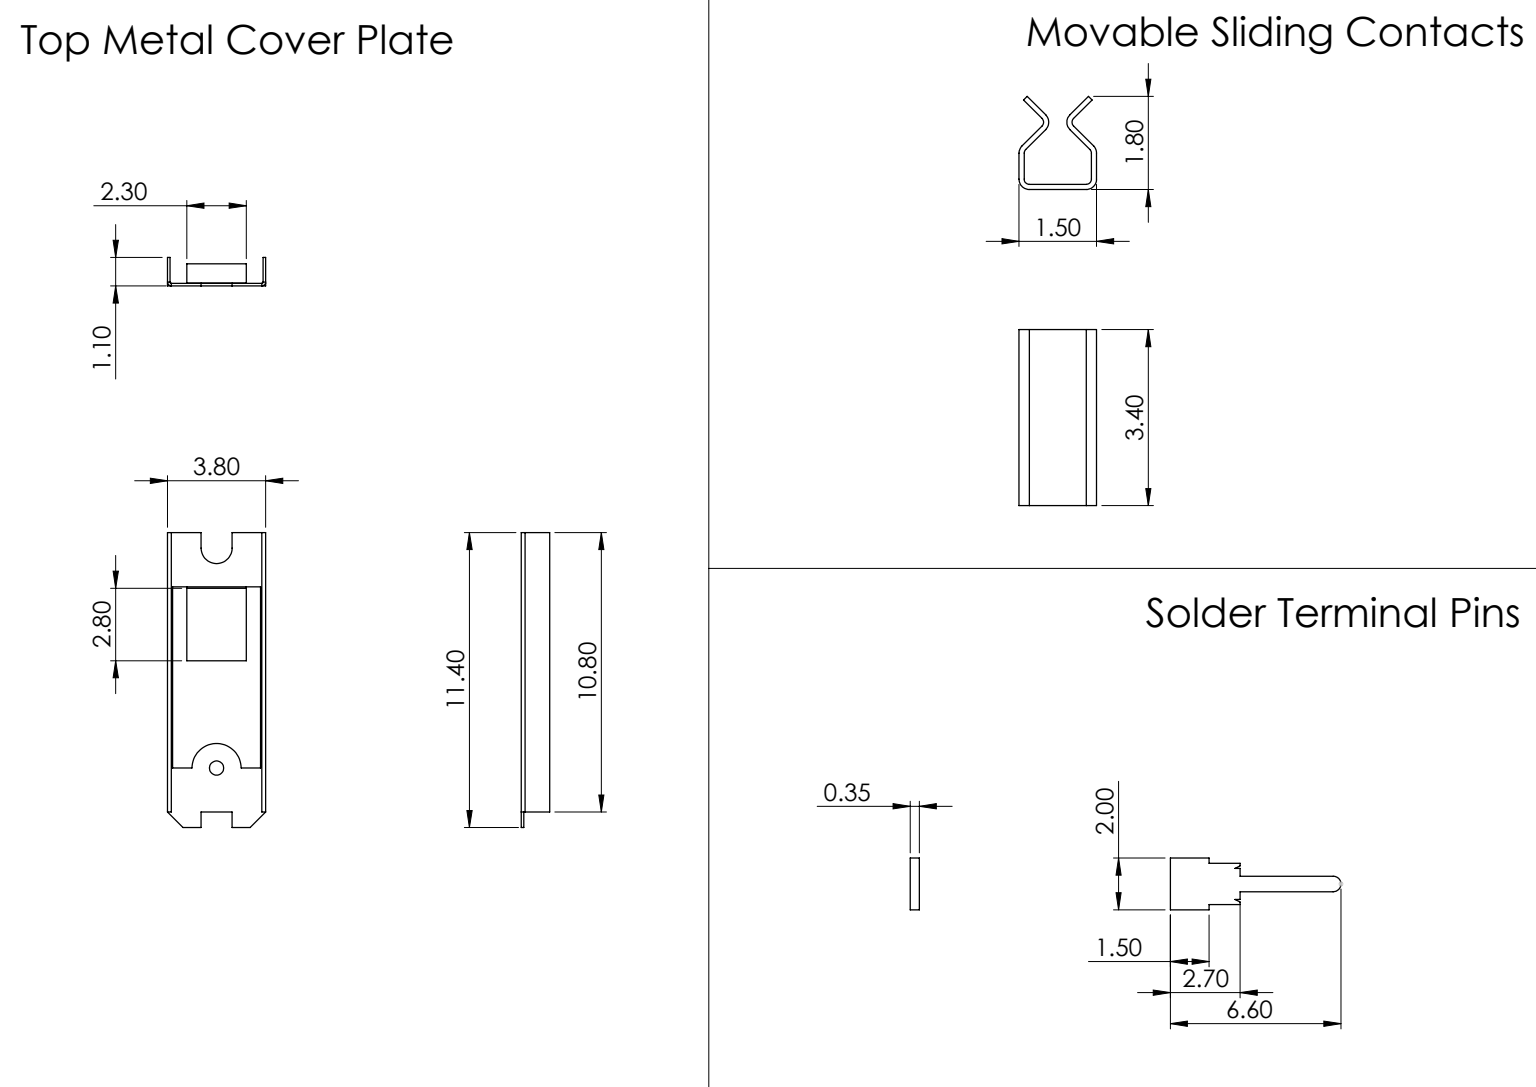
ISO-10303-21;
HEADER;
FILE_DESCRIPTION (('STEP AP214'),
    '1' );
FILE_NAME ('Solder Terminal Pins.step',
    '2026-10-09T19:32:29',
    ( '' ),
    ( '' ),
    'SwSTEP 2.0',
    'SolidWorks 2026',
    '' );
FILE_SCHEMA (( 'AUTOMOTIVE_DESIGN' ));
ENDSEC;

DATA;
#30=AXIS2_PLACEMENT_3D ( 'NONE', #13757, #16263, #2391 ) ;
#40=ORIENTED_EDGE ( 'NONE', *, *, #16715, .F. ) ;
#50=EDGE_LOOP ( 'NONE', ( #8387, #9597, #10554, #1667 ) ) ;
#66=ORIENTED_EDGE ( 'NONE', *, *, #5755, .T. ) ;
#103=VERTEX_POINT ( 'NONE', #12339 ) ;
#220=VECTOR ( 'NONE', #13007, 1000.000000000000000 ) ;
#244=APPLICATION_CONTEXT ( 'automotive_design' ) ;
#250=LINE ( 'NONE', #4404, #4362 ) ;
#296=CARTESIAN_POINT ( 'NONE',  ( 0.1749999999999999889, 8.800000000000000711, 0.4000000000000000222 ) ) ;
#310=ORIENTED_EDGE ( 'NONE', *, *, #13145, .F. ) ;
#326=ORIENTED_EDGE ( 'NONE', *, *, #6822, .T. ) ;
#331=VECTOR ( 'NONE', #11702, 1000.000000000000000 ) ;
#359=EDGE_CURVE ( 'NONE', #3082, #8454, #16331, .T. ) ;
#369=CARTESIAN_POINT ( 'NONE',  ( 0.1749999999999999889, 7.500000000000000000, 3.100000000000000089 ) ) ;
#450=VECTOR ( 'NONE', #504, 1000.000000000000000 ) ;
#504=DIRECTION ( 'NONE',  ( 5.551115123125779621E-17, 0.000000000000000000, 1.000000000000000000 ) ) ;
#537=CARTESIAN_POINT ( 'NONE',  ( -0.1749999999999999889, 8.200000000000001066, 0.4000000000000000222 ) ) ;
#551=DIRECTION ( 'NONE',  ( 0.000000000000000000, -1.000000000000000000, 0.000000000000000000 ) ) ;
#613=DIRECTION ( 'NONE',  ( 0.000000000000000000, 1.000000000000000000, 0.000000000000000000 ) ) ;
#646=CIRCLE ( 'NONE', #2745, 0.2999999999999999334 ) ;
#649=DIRECTION ( 'NONE',  ( -1.000000000000000000, 0.000000000000000000, 1.586032892321649771E-16 ) ) ;
#682=EDGE_CURVE ( 'NONE', #13202, #15500, #5739, .T. ) ;
#711=EDGE_CURVE ( 'NONE', #12486, #8493, #10165, .T. ) ;
#716=CARTESIAN_POINT ( 'NONE',  ( 0.1749999999999999889, 9.199999999999999289, 0.4000000000000000222 ) ) ;
#743=ORIENTED_EDGE ( 'NONE', *, *, #1591, .T. ) ;
#780=CARTESIAN_POINT ( 'NONE',  ( 0.1749999999999999889, 7.900000000000000355, 0.4000000000000000222 ) ) ;
#828=DIRECTION ( 'NONE',  ( 0.000000000000000000, 0.000000000000000000, -1.000000000000000000 ) ) ;
#853=SHAPE_REPRESENTATION ( 'Solder Terminal Pins', ( #17681 ), #4692 ) ;
#900=EDGE_LOOP ( 'NONE', ( #8185, #16443, #4602, #11112 ) ) ;
#904=FACE_OUTER_BOUND ( 'NONE', #4232, .T. ) ;
#915=CARTESIAN_POINT ( 'NONE',  ( 0.1749999999999999889, 9.500000000000000000, 3.100000000000000089 ) ) ;
#918=DIRECTION ( 'NONE',  ( -1.000000000000000000, 0.000000000000000000, 1.268826313857320014E-15 ) ) ;
#947=ADVANCED_FACE ( 'NONE', ( #4699 ), #14962, .T. ) ;
#953=ORIENTED_EDGE ( 'NONE', *, *, #17999, .F. ) ;
#959=VERTEX_POINT ( 'NONE', #2271 ) ;
#1067=FACE_OUTER_BOUND ( 'NONE', #7693, .T. ) ;
#1086=VECTOR ( 'NONE', #16477, 1000.000000000000000 ) ;
#1143=VECTOR ( 'NONE', #11238, 1000.000000000000000 ) ;
#1148=MECHANICAL_DESIGN_GEOMETRIC_PRESENTATION_REPRESENTATION('',(#6157),#4396);
#1164=PLANE ( 'NONE',  #16782 ) ;
#1218=PRODUCT_DEFINITION_CONTEXT ( 'detailed design', #244, 'design' ) ;
#1255=CARTESIAN_POINT ( 'NONE',  ( -0.1749999999999999889, 9.299999999999998934, 1.600000000000000089 ) ) ;
#1302=ORIENTED_EDGE ( 'NONE', *, *, #9005, .T. ) ;
#1311=CARTESIAN_POINT ( 'NONE',  ( -0.1749999999999999889, 7.700000000000000178, 1.600000000000000089 ) ) ;
#1333=DIRECTION ( 'NONE',  ( -6.167905692361979821E-17, 0.000000000000000000, -1.000000000000000000 ) ) ;
#1360=DIRECTION ( 'NONE',  ( -6.938893903907229610E-17, 0.000000000000000000, -1.000000000000000000 ) ) ;
#1389=VERTEX_POINT ( 'NONE', #15100 ) ;
#1403=CARTESIAN_POINT ( 'NONE',  ( -0.1749999999999999889, 8.200000000000001066, 0.4000000000000000222 ) ) ;
#1407=CARTESIAN_POINT ( 'NONE',  ( -0.1749999999999999889, 9.500000000000000000, 1.600000000000000089 ) ) ;
#1456=EDGE_LOOP ( 'NONE', ( #16915, #13820, #14175, #17317 ) ) ;
#1462=CARTESIAN_POINT ( 'NONE',  ( 0.1749999999999999889, 8.500000000000000000, -3.200000000000000178 ) ) ;
#1467=VECTOR ( 'NONE', #8980, 1000.000000000000000 ) ;
#1563=ORIENTED_EDGE ( 'NONE', *, *, #7259, .F. ) ;
#1568=ADVANCED_FACE ( 'NONE', ( #8498 ), #14148, .T. ) ;
#1591=EDGE_CURVE ( 'NONE', #4752, #1389, #4856, .T. ) ;
#1648=( LENGTH_UNIT ( ) NAMED_UNIT ( * ) SI_UNIT ( .MILLI., .METRE. ) );
#1667=ORIENTED_EDGE ( 'NONE', *, *, #711, .F. ) ;
#1669=ADVANCED_FACE ( 'NONE', ( #11908 ), #17176, .T. ) ;
#1693=ORIENTED_EDGE ( 'NONE', *, *, #17999, .T. ) ;
#1695=VECTOR ( 'NONE', #2486, 1000.000000000000114 ) ;
#1733=CARTESIAN_POINT ( 'NONE',  ( -0.1749999999999999889, 7.500000000000000000, 1.600000000000000089 ) ) ;
#1758=DIRECTION ( 'NONE',  ( -1.000000000000000000, 0.000000000000000000, 0.000000000000000000 ) ) ;
#1796=ORIENTED_EDGE ( 'NONE', *, *, #9182, .T. ) ;
#1803=CARTESIAN_POINT ( 'NONE',  ( -0.1749999999999999889, 7.799999999999999822, 0.4000000000000000222 ) ) ;
#1882=PLANE ( 'NONE',  #9376 ) ;
#1936=DIRECTION ( 'NONE',  ( 0.000000000000000000, 0.000000000000000000, -1.000000000000000000 ) ) ;
#1965=EDGE_LOOP ( 'NONE', ( #1302, #12791, #12438, #15138 ) ) ;
#2001=CARTESIAN_POINT ( 'NONE',  ( 0.1749999999999999889, 7.700000000000000178, 1.600000000000000089 ) ) ;
#2030=AXIS2_PLACEMENT_3D ( 'NONE', #6738, #13497, #12015 ) ;
#2031=LINE ( 'NONE', #13150, #5224 ) ;
#2052=VERTEX_POINT ( 'NONE', #11654 ) ;
#2094=ADVANCED_FACE ( 'NONE', ( #4882 ), #4704, .T. ) ;
#2101=LINE ( 'NONE', #9517, #11767 ) ;
#2139=CARTESIAN_POINT ( 'NONE',  ( -0.1749999999999999889, 9.199999999999999289, 0.4000000000000000222 ) ) ;
#2181=LINE ( 'NONE', #17608, #18254 ) ;
#2185=CARTESIAN_POINT ( 'NONE',  ( 0.1749999999999999889, 8.800000000000000711, -3.200000000000000178 ) ) ;
#2207=LINE ( 'NONE', #12020, #13126 ) ;
#2216=CARTESIAN_POINT ( 'NONE',  ( 0.1749999999999999889, 7.900000000000000355, 0.4000000000000000222 ) ) ;
#2232=LINE ( 'NONE', #13632, #3944 ) ;
#2271=CARTESIAN_POINT ( 'NONE',  ( 0.1749999999999999889, 9.500000000000000000, 3.100000000000000089 ) ) ;
#2273=DIRECTION ( 'NONE',  ( -1.000000000000000000, 0.000000000000000000, 0.000000000000000000 ) ) ;
#2345=VECTOR ( 'NONE', #6024, 1000.000000000000000 ) ;
#2391=DIRECTION ( 'NONE',  ( 0.000000000000000000, -1.000000000000000000, 0.000000000000000000 ) ) ;
#2414=EDGE_CURVE ( 'NONE', #11896, #13928, #2232, .T. ) ;
#2437=VERTEX_POINT ( 'NONE', #6771 ) ;
#2461=LINE ( 'NONE', #13744, #2914 ) ;
#2486=DIRECTION ( 'NONE',  ( 0.000000000000000000, -0.4472135954999567065, -0.8944271909999164105 ) ) ;
#2489=CARTESIAN_POINT ( 'NONE',  ( 0.1749999999999999889, 7.700000000000000178, 1.600000000000000089 ) ) ;
#2503=PLANE ( 'NONE',  #4069 ) ;
#2547=AXIS2_PLACEMENT_3D ( 'NONE', #17886, #15337, #3732 ) ;
#2567=LINE ( 'NONE', #16456, #17986 ) ;
#2569=EDGE_CURVE ( 'NONE', #8663, #9757, #2207, .T. ) ;
#2631=VECTOR ( 'NONE', #4875, 1000.000000000000000 ) ;
#2665=ORIENTED_EDGE ( 'NONE', *, *, #4156, .T. ) ;
#2745=AXIS2_PLACEMENT_3D ( 'NONE', #8071, #13711, #9339 ) ;
#2823=DIRECTION ( 'NONE',  ( 0.000000000000000000, -1.000000000000000000, 0.000000000000000000 ) ) ;
#2826=CARTESIAN_POINT ( 'NONE',  ( 0.1749999999999999889, 8.200000000000001066, 0.4000000000000000222 ) ) ;
#2834=CARTESIAN_POINT ( 'NONE',  ( 0.1749999999999999889, 9.500000000000000000, 1.600000000000000089 ) ) ;
#2914=VECTOR ( 'NONE', #5417, 1000.000000000000000 ) ;
#2920=ORIENTED_EDGE ( 'NONE', *, *, #5177, .T. ) ;
#2948=VERTEX_POINT ( 'NONE', #5196 ) ;
#2968=VECTOR ( 'NONE', #7672, 1000.000000000000000 ) ;
#3009=ORIENTED_EDGE ( 'NONE', *, *, #16003, .F. ) ;
#3015=ORIENTED_EDGE ( 'NONE', *, *, #9251, .T. ) ;
#3039=CARTESIAN_POINT ( 'NONE',  ( -0.1749999999999999889, 7.500000000000000000, 3.100000000000000089 ) ) ;
#3052=ADVANCED_FACE ( 'NONE', ( #5395 ), #11036, .T. ) ;
#3080=ORIENTED_EDGE ( 'NONE', *, *, #16715, .T. ) ;
#3081=LINE ( 'NONE', #5773, #1143 ) ;
#3082=VERTEX_POINT ( 'NONE', #1311 ) ;
#3092=CARTESIAN_POINT ( 'NONE',  ( 0.1749999999999999889, 7.700000000000000178, 0.4000000000000000222 ) ) ;
#3097=DIRECTION ( 'NONE',  ( 0.000000000000000000, -1.000000000000000000, 2.220446049250320181E-15 ) ) ;
#3108=ORIENTED_EDGE ( 'NONE', *, *, #16254, .F. ) ;
#3112=DIRECTION ( 'NONE',  ( -0.000000000000000000, 1.000000000000000000, 0.000000000000000000 ) ) ;
#3141=EDGE_CURVE ( 'NONE', #11906, #17304, #16772, .T. ) ;
#3300=ORIENTED_EDGE ( 'NONE', *, *, #9251, .F. ) ;
#3321=ORIENTED_EDGE ( 'NONE', *, *, #1591, .F. ) ;
#3325=PLANE ( 'NONE',  #10300 ) ;
#3402=CARTESIAN_POINT ( 'NONE',  ( -0.1749999999999999889, 8.800000000000000711, -3.200000000000000178 ) ) ;
#3415=CARTESIAN_POINT ( 'NONE',  ( 0.1749999999999999889, 9.099999999999999645, 0.4000000000000000222 ) ) ;
#3502=ORIENTED_EDGE ( 'NONE', *, *, #4388, .F. ) ;
#3506=VERTEX_POINT ( 'NONE', #2185 ) ;
#3517=ORIENTED_EDGE ( 'NONE', *, *, #5755, .F. ) ;
#3581=CARTESIAN_POINT ( 'NONE',  ( -0.1749999999999999889, 7.799999999999999822, 0.4000000000000000222 ) ) ;
#3597=CARTESIAN_POINT ( 'NONE',  ( 0.1749999999999999889, 7.700000000000000178, 0.4000000000000000222 ) ) ;
#3609=PLANE ( 'NONE',  #10566 ) ;
#3732=DIRECTION ( 'NONE',  ( 1.000000000000000000, 0.000000000000000000, 0.000000000000000000 ) ) ;
#3764=AXIS2_PLACEMENT_3D ( 'NONE', #16684, #6873, #14935 ) ;
#3812=LINE ( 'NONE', #6385, #11862 ) ;
#3831=DIRECTION ( 'NONE',  ( 0.000000000000000000, -1.000000000000000000, 0.000000000000000000 ) ) ;
#3867=LINE ( 'NONE', #3581, #4101 ) ;
#3874=FACE_OUTER_BOUND ( 'NONE', #13904, .T. ) ;
#3876=ORIENTED_EDGE ( 'NONE', *, *, #12580, .F. ) ;
#3924=FACE_OUTER_BOUND ( 'NONE', #11029, .T. ) ;
#3925=PLANE ( 'NONE',  #2547 ) ;
#3944=VECTOR ( 'NONE', #15120, 1000.000000000000000 ) ;
#4012=FACE_OUTER_BOUND ( 'NONE', #5869, .T. ) ;
#4069=AXIS2_PLACEMENT_3D ( 'NONE', #12224, #12136, #14814 ) ;
#4101=VECTOR ( 'NONE', #10628, 1000.000000000000000 ) ;
#4146=DIRECTION ( 'NONE',  ( 1.000000000000000000, 0.000000000000000000, 0.000000000000000000 ) ) ;
#4156=EDGE_CURVE ( 'NONE', #8493, #13928, #15310, .T. ) ;
#4159=CARTESIAN_POINT ( 'NONE',  ( 0.1749999999999999889, 7.799999999999999822, 0.4000000000000000222 ) ) ;
#4207=CARTESIAN_POINT ( 'NONE',  ( -0.1749999999999999889, 9.099999999999999645, 0.4000000000000000222 ) ) ;
#4222=CARTESIAN_POINT ( 'NONE',  ( 0.1749999999999999889, 8.800000000000000711, 0.4000000000000000222 ) ) ;
#4232=EDGE_LOOP ( 'NONE', ( #15122, #5278, #8292, #15026, #9377, #4506, #743, #9277, #4667, #10100, #2665, #17005, #5084, #11412, #1796, #2920, #6120, #18045 ) ) ;
#4256=AXIS2_PLACEMENT_3D ( 'NONE', #10529, #10355, #4985 ) ;
#4307=EDGE_CURVE ( 'NONE', #13650, #6378, #2031, .T. ) ;
#4311=DIRECTION ( 'NONE',  ( -1.000000000000000000, -9.028005242978079560E-48, 6.123233995736769734E-17 ) ) ;
#4347=AXIS2_PLACEMENT_3D ( 'NONE', #7837, #10710, #6726 ) ;
#4362=VECTOR ( 'NONE', #5889, 1000.000000000000000 ) ;
#4388=EDGE_CURVE ( 'NONE', #17710, #103, #12973, .T. ) ;
#4396=( GEOMETRIC_REPRESENTATION_CONTEXT ( 3 ) GLOBAL_UNCERTAINTY_ASSIGNED_CONTEXT ( ( #5299 ) ) GLOBAL_UNIT_ASSIGNED_CONTEXT ( ( #13099, #4837, #14651 ) ) REPRESENTATION_CONTEXT ( 'NONE', 'WORKASPACE' ) );
#4401=CARTESIAN_POINT ( 'NONE',  ( 0.1749999999999999889, 8.200000000000001066, -3.200000000000000178 ) ) ;
#4404=CARTESIAN_POINT ( 'NONE',  ( -0.1749999999999999889, 7.900000000000000355, 0.4000000000000000222 ) ) ;
#4441=CIRCLE ( 'NONE', #5631, 0.2999999999999999334 ) ;
#4470=DIRECTION ( 'NONE',  ( 6.938893903907229610E-17, 0.000000000000000000, 1.000000000000000000 ) ) ;
#4496=CARTESIAN_POINT ( 'NONE',  ( -0.1749999999999999889, 9.099999999999999645, 0.5999999999999999778 ) ) ;
#4506=ORIENTED_EDGE ( 'NONE', *, *, #5071, .T. ) ;
#4518=LINE ( 'NONE', #369, #2968 ) ;
#4554=CARTESIAN_POINT ( 'NONE',  ( 0.1749999999999999889, 9.299999999999998934, 0.4000000000000000222 ) ) ;
#4559=FILL_AREA_STYLE ('',( #15792 ) ) ;
#4568=CARTESIAN_POINT ( 'NONE',  ( 0.1749999999999999889, 7.799999999999999822, 0.4000000000000000222 ) ) ;
#4570=EDGE_CURVE ( 'NONE', #9728, #8493, #646, .T. ) ;
#4602=ORIENTED_EDGE ( 'NONE', *, *, #12870, .F. ) ;
#4615=PLANE ( 'NONE',  #6400 ) ;
#4667=ORIENTED_EDGE ( 'NONE', *, *, #15207, .T. ) ;
#4672=LINE ( 'NONE', #8934, #450 ) ;
#4692=( GEOMETRIC_REPRESENTATION_CONTEXT ( 3 ) GLOBAL_UNCERTAINTY_ASSIGNED_CONTEXT ( ( #9735 ) ) GLOBAL_UNIT_ASSIGNED_CONTEXT ( ( #1648, #11831, #15812 ) ) REPRESENTATION_CONTEXT ( 'NONE', 'WORKASPACE' ) );
#4699=FACE_OUTER_BOUND ( 'NONE', #15626, .T. ) ;
#4704=PLANE ( 'NONE',  #4256 ) ;
#4752=VERTEX_POINT ( 'NONE', #9901 ) ;
#4788=ORIENTED_EDGE ( 'NONE', *, *, #12474, .F. ) ;
#4807=VERTEX_POINT ( 'NONE', #780 ) ;
#4820=EDGE_CURVE ( 'NONE', #13610, #2948, #4672, .T. ) ;
#4837=( NAMED_UNIT ( * ) PLANE_ANGLE_UNIT ( ) SI_UNIT ( $, .RADIAN. ) );
#4856=LINE ( 'NONE', #4496, #15202 ) ;
#4875=DIRECTION ( 'NONE',  ( 0.000000000000000000, -1.000000000000000000, 0.000000000000000000 ) ) ;
#4882=FACE_OUTER_BOUND ( 'NONE', #900, .T. ) ;
#4899=DIRECTION ( 'NONE',  ( 0.000000000000000000, -0.4472135954999631458, 0.8944271909999133019 ) ) ;
#4917=VECTOR ( 'NONE', #14522, 1000.000000000000000 ) ;
#4972=AXIS2_PLACEMENT_3D ( 'NONE', #12151, #9355, #12576 ) ;
#4978=VECTOR ( 'NONE', #918, 1000.000000000000000 ) ;
#4985=DIRECTION ( 'NONE',  ( 1.000000000000000000, 0.000000000000000000, 0.000000000000000000 ) ) ;
#5045=ADVANCED_FACE ( 'NONE', ( #4012 ), #3925, .T. ) ;
#5071=EDGE_CURVE ( 'NONE', #6378, #4752, #2461, .T. ) ;
#5084=ORIENTED_EDGE ( 'NONE', *, *, #7259, .T. ) ;
#5099=AXIS2_PLACEMENT_3D ( 'NONE', #14607, #10698, #1758 ) ;
#5165=PLANE ( 'NONE',  #7988 ) ;
#5177=EDGE_CURVE ( 'NONE', #5929, #3082, #7182, .T. ) ;
#5191=LINE ( 'NONE', #3415, #15640 ) ;
#5196=CARTESIAN_POINT ( 'NONE',  ( 0.1749999999999999889, 7.500000000000000000, 3.100000000000000089 ) ) ;
#5224=VECTOR ( 'NONE', #16030, 1000.000000000000000 ) ;
#5230=ORIENTED_EDGE ( 'NONE', *, *, #15207, .F. ) ;
#5269=DIRECTION ( 'NONE',  ( 0.000000000000000000, 0.000000000000000000, -1.000000000000000000 ) ) ;
#5278=ORIENTED_EDGE ( 'NONE', *, *, #17844, .T. ) ;
#5299=UNCERTAINTY_MEASURE_WITH_UNIT (LENGTH_MEASURE( 1.000000000000000082E-05 ), #13099, 'distance_accuracy_value', 'NONE');
#5320=LINE ( 'NONE', #10966, #17668 ) ;
#5386=ORIENTED_EDGE ( 'NONE', *, *, #682, .T. ) ;
#5395=FACE_OUTER_BOUND ( 'NONE', #6299, .T. ) ;
#5417=DIRECTION ( 'NONE',  ( 0.000000000000000000, -0.4472135954999631458, 0.8944271909999133019 ) ) ;
#5434=DIRECTION ( 'NONE',  ( 0.000000000000000000, -0.4472135954999567065, -0.8944271909999164105 ) ) ;
#5469=EDGE_LOOP ( 'NONE', ( #7657, #8304, #15068, #310 ) ) ;
#5490=CARTESIAN_POINT ( 'NONE',  ( 0.1749999999999999889, 9.299999999999998934, 1.600000000000000089 ) ) ;
#5556=VECTOR ( 'NONE', #5656, 1000.000000000000000 ) ;
#5594=VECTOR ( 'NONE', #6045, 1000.000000000000000 ) ;
#5603=PLANE ( 'NONE',  #6994 ) ;
#5631=AXIS2_PLACEMENT_3D ( 'NONE', #10153, #17091, #613 ) ;
#5638=ORIENTED_EDGE ( 'NONE', *, *, #6822, .F. ) ;
#5656=DIRECTION ( 'NONE',  ( -1.000000000000000000, 0.000000000000000000, 0.000000000000000000 ) ) ;
#5700=DIRECTION ( 'NONE',  ( -1.000000000000000000, 0.000000000000000000, 1.586032892321649771E-16 ) ) ;
#5739=LINE ( 'NONE', #4159, #14373 ) ;
#5755=EDGE_CURVE ( 'NONE', #4807, #17154, #10546, .T. ) ;
#5773=CARTESIAN_POINT ( 'NONE',  ( 0.1749999999999999889, 9.500000000000000000, 1.600000000000000089 ) ) ;
#5793=ADVANCED_FACE ( 'NONE', ( #14718 ), #3609, .T. ) ;
#5869=EDGE_LOOP ( 'NONE', ( #14647, #12636, #10339, #11822 ) ) ;
#5889=DIRECTION ( 'NONE',  ( 0.000000000000000000, 0.000000000000000000, 1.000000000000000000 ) ) ;
#5894=LINE ( 'NONE', #1733, #6413 ) ;
#5901=DIRECTION ( 'NONE',  ( 0.000000000000000000, 0.000000000000000000, -1.000000000000000000 ) ) ;
#5929=VERTEX_POINT ( 'NONE', #17762 ) ;
#5980=DIRECTION ( 'NONE',  ( 0.000000000000000000, -1.000000000000000000, 0.000000000000000000 ) ) ;
#6024=DIRECTION ( 'NONE',  ( 0.000000000000000000, 1.000000000000000000, 2.220446049250309876E-16 ) ) ;
#6045=DIRECTION ( 'NONE',  ( -1.000000000000000000, 0.000000000000000000, 0.000000000000000000 ) ) ;
#6054=LINE ( 'NONE', #6147, #331 ) ;
#6076=ORIENTED_EDGE ( 'NONE', *, *, #14476, .F. ) ;
#6098=FACE_OUTER_BOUND ( 'NONE', #17094, .T. ) ;
#6120=ORIENTED_EDGE ( 'NONE', *, *, #359, .T. ) ;
#6147=CARTESIAN_POINT ( 'NONE',  ( 0.1749999999999999889, 7.700000000000000178, 1.600000000000000089 ) ) ;
#6157=STYLED_ITEM ( 'NONE', ( #14492 ), #8348 ) ;
#6299=EDGE_LOOP ( 'NONE', ( #15209, #12122, #12133, #12620 ) ) ;
#6331=ORIENTED_EDGE ( 'NONE', *, *, #11407, .F. ) ;
#6347=LINE ( 'NONE', #17912, #7046 ) ;
#6350=DIRECTION ( 'NONE',  ( 0.000000000000000000, 0.000000000000000000, 1.000000000000000000 ) ) ;
#6366=ORIENTED_EDGE ( 'NONE', *, *, #12580, .T. ) ;
#6378=VERTEX_POINT ( 'NONE', #2139 ) ;
#6385=CARTESIAN_POINT ( 'NONE',  ( 0.1749999999999999889, 9.500000000000000000, 3.100000000000000089 ) ) ;
#6390=EDGE_CURVE ( 'NONE', #6904, #1389, #5191, .T. ) ;
#6398=AXIS2_PLACEMENT_3D ( 'NONE', #1462, #4311, #14233 ) ;
#6400=AXIS2_PLACEMENT_3D ( 'NONE', #11664, #7502, #1936 ) ;
#6413=VECTOR ( 'NONE', #17796, 1000.000000000000000 ) ;
#6417=EDGE_CURVE ( 'NONE', #11376, #12725, #17237, .T. ) ;
#6463=VECTOR ( 'NONE', #11319, 1000.000000000000000 ) ;
#6560=DIRECTION ( 'NONE',  ( 0.000000000000000000, -1.000000000000000000, 0.000000000000000000 ) ) ;
#6676=LINE ( 'NONE', #18125, #8617 ) ;
#6694=VECTOR ( 'NONE', #15112, 1000.000000000000000 ) ;
#6726=DIRECTION ( 'NONE',  ( 0.000000000000000000, 1.000000000000000000, 0.000000000000000000 ) ) ;
#6738=CARTESIAN_POINT ( 'NONE',  ( 0.1749999999999999889, 5.000000000000000000, -1.071565949253929989E-17 ) ) ;
#6771=CARTESIAN_POINT ( 'NONE',  ( 0.1749999999999999889, 9.299999999999998934, 0.4000000000000000222 ) ) ;
#6774=ADVANCED_FACE ( 'NONE', ( #904 ), #17812, .T. ) ;
#6822=EDGE_CURVE ( 'NONE', #16560, #13202, #8210, .T. ) ;
#6831=VECTOR ( 'NONE', #8481, 1000.000000000000000 ) ;
#6873=DIRECTION ( 'NONE',  ( -1.586032892321649771E-16, 0.000000000000000000, -1.000000000000000000 ) ) ;
#6892=LINE ( 'NONE', #14106, #17605 ) ;
#6904=VERTEX_POINT ( 'NONE', #15253 ) ;
#6981=CARTESIAN_POINT ( 'NONE',  ( 0.1749999999999999889, 7.700000000000000178, 1.600000000000000089 ) ) ;
#6994=AXIS2_PLACEMENT_3D ( 'NONE', #6981, #11054, #2823 ) ;
#7015=FACE_OUTER_BOUND ( 'NONE', #5469, .T. ) ;
#7031=PLANE ( 'NONE',  #4972 ) ;
#7046=VECTOR ( 'NONE', #10911, 1000.000000000000000 ) ;
#7182=LINE ( 'NONE', #8652, #12641 ) ;
#7230=ORIENTED_EDGE ( 'NONE', *, *, #10357, .F. ) ;
#7259=EDGE_CURVE ( 'NONE', #17154, #2052, #250, .T. ) ;
#7268=DIRECTION ( 'NONE',  ( 0.000000000000000000, -2.220446049250320181E-15, -1.000000000000000000 ) ) ;
#7278=ORIENTED_EDGE ( 'NONE', *, *, #16387, .F. ) ;
#7372=SURFACE_SIDE_STYLE ('',( #17240 ) ) ;
#7502=DIRECTION ( 'NONE',  ( 0.000000000000000000, -1.000000000000000000, 0.000000000000000000 ) ) ;
#7577=VECTOR ( 'NONE', #17418, 1000.000000000000000 ) ;
#7607=CARTESIAN_POINT ( 'NONE',  ( 0.1749999999999999889, 9.099999999999999645, 0.5999999999999999778 ) ) ;
#7657=ORIENTED_EDGE ( 'NONE', *, *, #11407, .T. ) ;
#7672=DIRECTION ( 'NONE',  ( -1.000000000000000000, 0.000000000000000000, 0.000000000000000000 ) ) ;
#7693=EDGE_LOOP ( 'NONE', ( #12595, #66, #9346, #13675 ) ) ;
#7734=CARTESIAN_POINT ( 'NONE',  ( -0.1749999999999999889, 9.299999999999998934, 0.4000000000000000222 ) ) ;
#7760=LINE ( 'NONE', #2489, #2631 ) ;
#7821=ADVANCED_FACE ( 'NONE', ( #14709 ), #2503, .T. ) ;
#7837=CARTESIAN_POINT ( 'NONE',  ( -0.1749999999999999889, 5.000000000000000000, 1.071565949253929989E-17 ) ) ;
#7850=CARTESIAN_POINT ( 'NONE',  ( 0.1749999999999999889, 7.799999999999999822, 0.4000000000000000222 ) ) ;
#7988=AXIS2_PLACEMENT_3D ( 'NONE', #15101, #6560, #5269 ) ;
#8013=CARTESIAN_POINT ( 'NONE',  ( -0.1749999999999999889, 7.700000000000000178, 1.600000000000000089 ) ) ;
#8071=CARTESIAN_POINT ( 'NONE',  ( -0.1749999999999999889, 8.500000000000000000, -3.200000000000000178 ) ) ;
#8185=ORIENTED_EDGE ( 'NONE', *, *, #13318, .T. ) ;
#8210=LINE ( 'NONE', #18087, #14396 ) ;
#8292=ORIENTED_EDGE ( 'NONE', *, *, #3141, .T. ) ;
#8304=ORIENTED_EDGE ( 'NONE', *, *, #711, .T. ) ;
#8348=MANIFOLD_SOLID_BREP ( 'Stock-MAS-687-1', #14386 ) ;
#8360=DIRECTION ( 'NONE',  ( 0.000000000000000000, -1.000000000000000000, 0.000000000000000000 ) ) ;
#8369=ORIENTED_EDGE ( 'NONE', *, *, #6390, .T. ) ;
#8387=ORIENTED_EDGE ( 'NONE', *, *, #11852, .T. ) ;
#8411=DIRECTION ( 'NONE',  ( 0.000000000000000000, -1.000000000000000000, -2.220446049250309876E-16 ) ) ;
#8454=VERTEX_POINT ( 'NONE', #13054 ) ;
#8465=EDGE_LOOP ( 'NONE', ( #3080, #8369, #3321, #10212 ) ) ;
#8481=DIRECTION ( 'NONE',  ( -1.000000000000000000, 0.000000000000000000, 0.000000000000000000 ) ) ;
#8493=VERTEX_POINT ( 'NONE', #15572 ) ;
#8498=FACE_OUTER_BOUND ( 'NONE', #1965, .T. ) ;
#8617=VECTOR ( 'NONE', #13724, 1000.000000000000000 ) ;
#8652=CARTESIAN_POINT ( 'NONE',  ( -0.1749999999999999889, 7.700000000000000178, 0.4000000000000000222 ) ) ;
#8663=VERTEX_POINT ( 'NONE', #3597 ) ;
#8667=AXIS2_PLACEMENT_3D ( 'NONE', #9702, #15369, #8411 ) ;
#8693=ADVANCED_FACE ( 'NONE', ( #6098 ), #3325, .T. ) ;
#8740=LINE ( 'NONE', #14384, #220 ) ;
#8745=APPLICATION_CONTEXT ( 'automotive_design' ) ;
#8746=VECTOR ( 'NONE', #9485, 1000.000000000000000 ) ;
#8764=DIRECTION ( 'NONE',  ( 1.000000000000000000, 0.000000000000000000, 0.000000000000000000 ) ) ;
#8795=ORIENTED_EDGE ( 'NONE', *, *, #15544, .F. ) ;
#8823=ORIENTED_EDGE ( 'NONE', *, *, #4820, .F. ) ;
#8934=CARTESIAN_POINT ( 'NONE',  ( 0.1749999999999999889, 7.500000000000000000, 1.600000000000000089 ) ) ;
#8937=EDGE_CURVE ( 'NONE', #8663, #5929, #15783, .T. ) ;
#8939=LINE ( 'NONE', #16935, #5556 ) ;
#8980=DIRECTION ( 'NONE',  ( 0.000000000000000000, -1.000000000000000000, 2.220446049250320181E-15 ) ) ;
#9005=EDGE_CURVE ( 'NONE', #2948, #959, #10023, .T. ) ;
#9043=EDGE_CURVE ( 'NONE', #11376, #6378, #13064, .T. ) ;
#9079=VECTOR ( 'NONE', #649, 1000.000000000000000 ) ;
#9182=EDGE_CURVE ( 'NONE', #15500, #5929, #3867, .T. ) ;
#9209=ADVANCED_FACE ( 'NONE', ( #13768 ), #17822, .F. ) ;
#9248=EDGE_CURVE ( 'NONE', #959, #16239, #16276, .T. ) ;
#9251=EDGE_CURVE ( 'NONE', #4807, #16560, #2567, .T. ) ;
#9277=ORIENTED_EDGE ( 'NONE', *, *, #17389, .T. ) ;
#9339=DIRECTION ( 'NONE',  ( 0.000000000000000000, 1.000000000000000000, 0.000000000000000000 ) ) ;
#9346=ORIENTED_EDGE ( 'NONE', *, *, #15827, .F. ) ;
#9355=DIRECTION ( 'NONE',  ( 1.368455531567199917E-48, 1.000000000000000000, 1.233581138472399909E-16 ) ) ;
#9376=AXIS2_PLACEMENT_3D ( 'NONE', #4554, #7268, #3097 ) ;
#9377=ORIENTED_EDGE ( 'NONE', *, *, #4307, .T. ) ;
#9384=VECTOR ( 'NONE', #8360, 1000.000000000000000 ) ;
#9413=AXIS2_PLACEMENT_3D ( 'NONE', #16611, #9476, #3831 ) ;
#9441=ORIENTED_EDGE ( 'NONE', *, *, #16967, .T. ) ;
#9461=ORIENTED_EDGE ( 'NONE', *, *, #15614, .F. ) ;
#9476=DIRECTION ( 'NONE',  ( 0.000000000000000000, 0.000000000000000000, -1.000000000000000000 ) ) ;
#9485=DIRECTION ( 'NONE',  ( 0.000000000000000000, -1.000000000000000000, 0.000000000000000000 ) ) ;
#9517=CARTESIAN_POINT ( 'NONE',  ( 0.1749999999999999889, 8.200000000000001066, 0.4000000000000000222 ) ) ;
#9521=ORIENTED_EDGE ( 'NONE', *, *, #17153, .T. ) ;
#9597=ORIENTED_EDGE ( 'NONE', *, *, #2414, .T. ) ;
#9702=CARTESIAN_POINT ( 'NONE',  ( 0.1749999999999999889, 7.500000000000000000, 3.100000000000000089 ) ) ;
#9728=VERTEX_POINT ( 'NONE', #3402 ) ;
#9735=UNCERTAINTY_MEASURE_WITH_UNIT (LENGTH_MEASURE( 1.000000000000000082E-05 ), #1648, 'distance_accuracy_value', 'NONE');
#9757=VERTEX_POINT ( 'NONE', #2001 ) ;
#9802=PRODUCT_DEFINITION_SHAPE ( 'NONE', 'NONE',  #14462 ) ;
#9867=DIRECTION ( 'NONE',  ( 0.000000000000000000, -1.000000000000000000, 0.000000000000000000 ) ) ;
#9901=CARTESIAN_POINT ( 'NONE',  ( -0.1749999999999999889, 9.099999999999999645, 0.5999999999999999778 ) ) ;
#9950=LINE ( 'NONE', #12633, #16478 ) ;
#9975=LINE ( 'NONE', #4222, #10539 ) ;
#10001=DIRECTION ( 'NONE',  ( -1.000000000000000000, 0.000000000000000000, 0.000000000000000000 ) ) ;
#10013=VECTOR ( 'NONE', #11316, 1000.000000000000000 ) ;
#10023=LINE ( 'NONE', #17035, #2345 ) ;
#10084=ORIENTED_EDGE ( 'NONE', *, *, #682, .F. ) ;
#10100=ORIENTED_EDGE ( 'NONE', *, *, #4570, .T. ) ;
#10119=ORIENTED_EDGE ( 'NONE', *, *, #9043, .T. ) ;
#10131=FACE_OUTER_BOUND ( 'NONE', #14198, .T. ) ;
#10153=CARTESIAN_POINT ( 'NONE',  ( 0.1749999999999999889, 8.500000000000000000, -3.200000000000000178 ) ) ;
#10165=LINE ( 'NONE', #14062, #14652 ) ;
#10212=ORIENTED_EDGE ( 'NONE', *, *, #15608, .F. ) ;
#10213=CARTESIAN_POINT ( 'NONE',  ( 0.1749999999999999889, 8.200000000000001066, -3.200000000000000178 ) ) ;
#10214=SURFACE_STYLE_USAGE ( .BOTH. , #7372 ) ;
#10300=AXIS2_PLACEMENT_3D ( 'NONE', #2216, #551, #828 ) ;
#10339=ORIENTED_EDGE ( 'NONE', *, *, #17844, .F. ) ;
#10355=DIRECTION ( 'NONE',  ( -0.000000000000000000, 1.000000000000000000, 0.000000000000000000 ) ) ;
#10357=EDGE_CURVE ( 'NONE', #2437, #11376, #17402, .T. ) ;
#10481=ORIENTED_EDGE ( 'NONE', *, *, #9182, .F. ) ;
#10529=CARTESIAN_POINT ( 'NONE',  ( 0.1749999999999999889, 9.299999999999998934, 1.600000000000000089 ) ) ;
#10539=VECTOR ( 'NONE', #14041, 1000.000000000000000 ) ;
#10546=LINE ( 'NONE', #14822, #9079 ) ;
#10554=ORIENTED_EDGE ( 'NONE', *, *, #4156, .F. ) ;
#10566=AXIS2_PLACEMENT_3D ( 'NONE', #17483, #12143, #17563 ) ;
#10628=DIRECTION ( 'NONE',  ( 0.000000000000000000, -1.000000000000000000, 0.000000000000000000 ) ) ;
#10632=CARTESIAN_POINT ( 'NONE',  ( 0.1749999999999999889, 8.800000000000000711, -3.200000000000000178 ) ) ;
#10681=CARTESIAN_POINT ( 'NONE',  ( 0.1749999999999999889, 8.200000000000001066, 0.4000000000000000222 ) ) ;
#10698=DIRECTION ( 'NONE',  ( 0.000000000000000000, 0.8944271909999159664, -0.4472135954999579832 ) ) ;
#10710=DIRECTION ( 'NONE',  ( -1.000000000000000000, 0.000000000000000000, 6.123233995736769734E-17 ) ) ;
#10737=EDGE_CURVE ( 'NONE', #2948, #12005, #4518, .T. ) ;
#10867=FACE_OUTER_BOUND ( 'NONE', #17313, .T. ) ;
#10901=FACE_OUTER_BOUND ( 'NONE', #15963, .T. ) ;
#10911=DIRECTION ( 'NONE',  ( 0.000000000000000000, 1.000000000000000000, 2.220446049250309876E-16 ) ) ;
#10940=ADVANCED_FACE ( 'NONE', ( #3874 ), #5165, .T. ) ;
#10966=CARTESIAN_POINT ( 'NONE',  ( -0.1749999999999999889, 9.500000000000000000, 3.100000000000000089 ) ) ;
#10971=ORIENTED_EDGE ( 'NONE', *, *, #9043, .F. ) ;
#11002=LINE ( 'NONE', #18098, #14155 ) ;
#11029=EDGE_LOOP ( 'NONE', ( #11680, #9441, #11890, #3876 ) ) ;
#11036=PLANE ( 'NONE',  #3764 ) ;
#11054=DIRECTION ( 'NONE',  ( 0.000000000000000000, 0.000000000000000000, -1.000000000000000000 ) ) ;
#11059=DIRECTION ( 'NONE',  ( 0.000000000000000000, 0.000000000000000000, -1.000000000000000000 ) ) ;
#11091=ORIENTED_EDGE ( 'NONE', *, *, #5177, .F. ) ;
#11112=ORIENTED_EDGE ( 'NONE', *, *, #13683, .F. ) ;
#11137=ORIENTED_EDGE ( 'NONE', *, *, #13145, .T. ) ;
#11191=CARTESIAN_POINT ( 'NONE',  ( 0.000000000000000000, 0.000000000000000000, 0.000000000000000000 ) ) ;
#11222=CARTESIAN_POINT ( 'NONE',  ( -0.1749999999999999889, 8.200000000000001066, -3.200000000000000178 ) ) ;
#11238=DIRECTION ( 'NONE',  ( 0.000000000000000000, -1.000000000000000000, 0.000000000000000000 ) ) ;
#11297=ADVANCED_BREP_SHAPE_REPRESENTATION ( '', ( #8348, #17681 ), #4692 ) ;
#11316=DIRECTION ( 'NONE',  ( 6.167905692361979821E-17, 0.000000000000000000, 1.000000000000000000 ) ) ;
#11319=DIRECTION ( 'NONE',  ( -1.000000000000000000, 0.000000000000000000, 0.000000000000000000 ) ) ;
#11348=LINE ( 'NONE', #4207, #17953 ) ;
#11376=VERTEX_POINT ( 'NONE', #14672 ) ;
#11389=ORIENTED_EDGE ( 'NONE', *, *, #15608, .T. ) ;
#11407=EDGE_CURVE ( 'NONE', #3506, #12486, #4441, .T. ) ;
#11412=ORIENTED_EDGE ( 'NONE', *, *, #16003, .T. ) ;
#11487=ORIENTED_EDGE ( 'NONE', *, *, #13318, .F. ) ;
#11560=DIRECTION ( 'NONE',  ( -1.000000000000000000, 0.000000000000000000, 0.000000000000000000 ) ) ;
#11636=SHAPE_REPRESENTATION_RELATIONSHIP ( 'NONE' , 'NONE' ,  #853, #11297 ) ;
#11654=CARTESIAN_POINT ( 'NONE',  ( -0.1749999999999999889, 7.900000000000000355, 0.5999999999999999778 ) ) ;
#11664=CARTESIAN_POINT ( 'NONE',  ( 0.1749999999999999889, 8.200000000000001066, -3.200000000000000178 ) ) ;
#11680=ORIENTED_EDGE ( 'NONE', *, *, #13100, .T. ) ;
#11699=LINE ( 'NONE', #10213, #15108 ) ;
#11702=DIRECTION ( 'NONE',  ( -1.000000000000000000, 0.000000000000000000, 0.000000000000000000 ) ) ;
#11767=VECTOR ( 'NONE', #12116, 1000.000000000000000 ) ;
#11797=CARTESIAN_POINT ( 'NONE',  ( 0.1749999999999999889, 9.299999999999998934, 0.4000000000000000222 ) ) ;
#11822=ORIENTED_EDGE ( 'NONE', *, *, #12842, .F. ) ;
#11831=( NAMED_UNIT ( * ) PLANE_ANGLE_UNIT ( ) SI_UNIT ( $, .RADIAN. ) );
#11852=EDGE_CURVE ( 'NONE', #12486, #11896, #11699, .T. ) ;
#11862=VECTOR ( 'NONE', #12057, 1000.000000000000000 ) ;
#11872=ORIENTED_EDGE ( 'NONE', *, *, #13100, .F. ) ;
#11890=ORIENTED_EDGE ( 'NONE', *, *, #359, .F. ) ;
#11896=VERTEX_POINT ( 'NONE', #10681 ) ;
#11906=VERTEX_POINT ( 'NONE', #14942 ) ;
#11908=FACE_OUTER_BOUND ( 'NONE', #8465, .T. ) ;
#12005=VERTEX_POINT ( 'NONE', #3039 ) ;
#12015=DIRECTION ( 'NONE',  ( 0.000000000000000000, 1.000000000000000000, 0.000000000000000000 ) ) ;
#12020=CARTESIAN_POINT ( 'NONE',  ( 0.1749999999999999889, 7.700000000000000178, 0.4000000000000000222 ) ) ;
#12057=DIRECTION ( 'NONE',  ( -1.000000000000000000, 0.000000000000000000, 0.000000000000000000 ) ) ;
#12116=DIRECTION ( 'NONE',  ( 0.000000000000000000, -1.000000000000000000, 0.000000000000000000 ) ) ;
#12122=ORIENTED_EDGE ( 'NONE', *, *, #4388, .T. ) ;
#12133=ORIENTED_EDGE ( 'NONE', *, *, #17389, .F. ) ;
#12136=DIRECTION ( 'NONE',  ( -7.092954723563668294E-17, -0.8944271909999148562, -0.4472135954999599261 ) ) ;
#12143=DIRECTION ( 'NONE',  ( 0.000000000000000000, -1.000000000000000000, 0.000000000000000000 ) ) ;
#12151=CARTESIAN_POINT ( 'NONE',  ( 0.1749999999999999889, 8.800000000000000711, 0.4000000000000000222 ) ) ;
#12155=PRODUCT_CONTEXT ( 'NONE', #8745, 'mechanical' ) ;
#12224=CARTESIAN_POINT ( 'NONE',  ( 0.1749999999999999889, 9.199999999999999289, 0.4000000000000000222 ) ) ;
#12239=FACE_OUTER_BOUND ( 'NONE', #13869, .T. ) ;
#12292=ADVANCED_FACE ( 'NONE', ( #10901 ), #16637, .T. ) ;
#12339=CARTESIAN_POINT ( 'NONE',  ( -0.1749999999999999889, 8.800000000000000711, 0.4000000000000000222 ) ) ;
#12411=LINE ( 'NONE', #14740, #6694 ) ;
#12438=ORIENTED_EDGE ( 'NONE', *, *, #14488, .F. ) ;
#12467=LINE ( 'NONE', #2834, #6831 ) ;
#12474=EDGE_CURVE ( 'NONE', #16239, #11906, #12467, .T. ) ;
#12486=VERTEX_POINT ( 'NONE', #4401 ) ;
#12576=DIRECTION ( 'NONE',  ( 0.000000000000000000, 1.233581138472399909E-16, -1.000000000000000000 ) ) ;
#12580=EDGE_CURVE ( 'NONE', #9757, #3082, #6054, .T. ) ;
#12595=ORIENTED_EDGE ( 'NONE', *, *, #14476, .T. ) ;
#12620=ORIENTED_EDGE ( 'NONE', *, *, #6390, .F. ) ;
#12633=CARTESIAN_POINT ( 'NONE',  ( 0.1749999999999999889, 9.099999999999999645, 0.5999999999999999778 ) ) ;
#12636=ORIENTED_EDGE ( 'NONE', *, *, #12474, .T. ) ;
#12641=VECTOR ( 'NONE', #4470, 1000.000000000000000 ) ;
#12712=PRODUCT_DEFINITION_FORMATION_WITH_SPECIFIED_SOURCE ( 'ANY', '', #13935, .NOT_KNOWN. ) ;
#12725=VERTEX_POINT ( 'NONE', #7607 ) ;
#12751=ORIENTED_EDGE ( 'NONE', *, *, #8937, .F. ) ;
#12791=ORIENTED_EDGE ( 'NONE', *, *, #12842, .T. ) ;
#12842=EDGE_CURVE ( 'NONE', #959, #13844, #3812, .T. ) ;
#12870=EDGE_CURVE ( 'NONE', #17304, #13650, #6676, .T. ) ;
#12904=VECTOR ( 'NONE', #13239, 1000.000000000000000 ) ;
#12971=FACE_OUTER_BOUND ( 'NONE', #50, .T. ) ;
#12973=LINE ( 'NONE', #296, #12904 ) ;
#13007=DIRECTION ( 'NONE',  ( -1.000000000000000000, 0.000000000000000000, 0.000000000000000000 ) ) ;
#13033=ORIENTED_EDGE ( 'NONE', *, *, #9248, .F. ) ;
#13054=CARTESIAN_POINT ( 'NONE',  ( -0.1749999999999999889, 7.500000000000000000, 1.600000000000000089 ) ) ;
#13064=LINE ( 'NONE', #716, #6463 ) ;
#13099=( LENGTH_UNIT ( ) NAMED_UNIT ( * ) SI_UNIT ( .MILLI., .METRE. ) );
#13100=EDGE_CURVE ( 'NONE', #9757, #13610, #7760, .T. ) ;
#13126=VECTOR ( 'NONE', #17743, 1000.000000000000000 ) ;
#13145=EDGE_CURVE ( 'NONE', #3506, #9728, #17742, .T. ) ;
#13150=CARTESIAN_POINT ( 'NONE',  ( -0.1749999999999999889, 9.299999999999998934, 0.4000000000000000222 ) ) ;
#13202=VERTEX_POINT ( 'NONE', #7850 ) ;
#13239=DIRECTION ( 'NONE',  ( -1.000000000000000000, 0.000000000000000000, 1.586032892321649771E-16 ) ) ;
#13296=ORIENTED_EDGE ( 'NONE', *, *, #3141, .F. ) ;
#13318=EDGE_CURVE ( 'NONE', #17967, #2437, #11002, .T. ) ;
#13340=DIRECTION ( 'NONE',  ( -1.000000000000000000, 0.000000000000000000, 1.586032892321649771E-16 ) ) ;
#13354=LINE ( 'NONE', #16666, #1086 ) ;
#13469=CARTESIAN_POINT ( 'NONE',  ( -0.1749999999999999889, 7.900000000000000355, 0.4000000000000000222 ) ) ;
#13496=LINE ( 'NONE', #13767, #1695 ) ;
#13497=DIRECTION ( 'NONE',  ( -1.000000000000000000, 0.000000000000000000, 6.123233995736769734E-17 ) ) ;
#13610=VERTEX_POINT ( 'NONE', #17895 ) ;
#13632=CARTESIAN_POINT ( 'NONE',  ( 0.1749999999999999889, 8.200000000000001066, 0.4000000000000000222 ) ) ;
#13650=VERTEX_POINT ( 'NONE', #7734 ) ;
#13651=DIRECTION ( 'NONE',  ( -9.251858538542969116E-17, 0.000000000000000000, -1.000000000000000000 ) ) ;
#13675=ORIENTED_EDGE ( 'NONE', *, *, #2414, .F. ) ;
#13680=ADVANCED_FACE ( 'NONE', ( #10131 ), #1882, .T. ) ;
#13683=EDGE_CURVE ( 'NONE', #17967, #17304, #8740, .T. ) ;
#13692=DIRECTION ( 'NONE',  ( -5.551115123125779621E-17, 0.000000000000000000, -1.000000000000000000 ) ) ;
#13711=DIRECTION ( 'NONE',  ( -1.000000000000000000, 0.000000000000000000, 6.123233995736769734E-17 ) ) ;
#13724=DIRECTION ( 'NONE',  ( -6.938893903907229610E-17, 0.000000000000000000, -1.000000000000000000 ) ) ;
#13744=CARTESIAN_POINT ( 'NONE',  ( -0.1749999999999999889, 9.199999999999999289, 0.4000000000000000222 ) ) ;
#13757=CARTESIAN_POINT ( 'NONE',  ( 0.1749999999999999889, 9.500000000000000000, 1.600000000000000089 ) ) ;
#13767=CARTESIAN_POINT ( 'NONE',  ( -0.1749999999999999889, 7.900000000000000355, 0.5999999999999999778 ) ) ;
#13768=FACE_OUTER_BOUND ( 'NONE', #15274, .T. ) ;
#13820=ORIENTED_EDGE ( 'NONE', *, *, #10737, .T. ) ;
#13844=VERTEX_POINT ( 'NONE', #15407 ) ;
#13869=EDGE_LOOP ( 'NONE', ( #15215, #11137, #5230, #3502 ) ) ;
#13904=EDGE_LOOP ( 'NONE', ( #17856, #6366, #11091, #12751 ) ) ;
#13928=VERTEX_POINT ( 'NONE', #1403 ) ;
#13935=PRODUCT ( 'Solder Terminal Pins', 'Solder Terminal Pins', '', ( #12155 ) ) ;
#14041=DIRECTION ( 'NONE',  ( -6.167905692361979821E-17, 0.000000000000000000, -1.000000000000000000 ) ) ;
#14062=CARTESIAN_POINT ( 'NONE',  ( 0.1749999999999999889, 8.200000000000001066, -3.200000000000000178 ) ) ;
#14098=ADVANCED_FACE ( 'NONE', ( #12971 ), #4615, .T. ) ;
#14106=CARTESIAN_POINT ( 'NONE',  ( -0.1749999999999999889, 8.800000000000000711, 0.4000000000000000222 ) ) ;
#14141=CYLINDRICAL_SURFACE ( 'NONE', #6398, 0.2999999999999999334 ) ;
#14148=PLANE ( 'NONE',  #8667 ) ;
#14155=VECTOR ( 'NONE', #1360, 1000.000000000000000 ) ;
#14175=ORIENTED_EDGE ( 'NONE', *, *, #16496, .F. ) ;
#14198=EDGE_LOOP ( 'NONE', ( #14341, #10119, #17118, #8795 ) ) ;
#14233=DIRECTION ( 'NONE',  ( 0.000000000000000000, 1.000000000000000000, 0.000000000000000000 ) ) ;
#14341=ORIENTED_EDGE ( 'NONE', *, *, #10357, .T. ) ;
#14373=VECTOR ( 'NONE', #11560, 1000.000000000000000 ) ;
#14384=CARTESIAN_POINT ( 'NONE',  ( 0.1749999999999999889, 9.299999999999998934, 1.600000000000000089 ) ) ;
#14386=CLOSED_SHELL ( 'NONE', ( #12292, #2094, #13680, #7821, #1669, #3052, #18255, #16279, #14098, #16781, #8693, #947, #17867, #10940, #15281, #5793, #6774, #5045, #9209, #1568 ) ) ;
#14396=VECTOR ( 'NONE', #5434, 1000.000000000000114 ) ;
#14462=PRODUCT_DEFINITION ( 'UNKNOWN', '', #12712, #1218 ) ;
#14476=EDGE_CURVE ( 'NONE', #11896, #4807, #2101, .T. ) ;
#14488=EDGE_CURVE ( 'NONE', #12005, #13844, #6347, .T. ) ;
#14492=PRESENTATION_STYLE_ASSIGNMENT (( #10214 ) ) ;
#14522=DIRECTION ( 'NONE',  ( 0.000000000000000000, -1.000000000000000000, 0.000000000000000000 ) ) ;
#14607=CARTESIAN_POINT ( 'NONE',  ( 0.1749999999999999889, 7.900000000000000355, 0.5999999999999999778 ) ) ;
#14637=SHAPE_DEFINITION_REPRESENTATION ( #9802, #853 ) ;
#14647=ORIENTED_EDGE ( 'NONE', *, *, #9248, .T. ) ;
#14651=( NAMED_UNIT ( * ) SI_UNIT ( $, .STERADIAN. ) SOLID_ANGLE_UNIT ( ) );
#14652=VECTOR ( 'NONE', #10001, 1000.000000000000000 ) ;
#14671=VECTOR ( 'NONE', #4899, 1000.000000000000000 ) ;
#14672=CARTESIAN_POINT ( 'NONE',  ( 0.1749999999999999889, 9.199999999999999289, 0.4000000000000000222 ) ) ;
#14709=FACE_OUTER_BOUND ( 'NONE', #15800, .T. ) ;
#14718=FACE_OUTER_BOUND ( 'NONE', #1456, .T. ) ;
#14740=CARTESIAN_POINT ( 'NONE',  ( 0.1749999999999999889, 9.099999999999999645, 0.5999999999999999778 ) ) ;
#14814=DIRECTION ( 'NONE',  ( 0.000000000000000000, 0.4472135954999599261, -0.8944271909999148562 ) ) ;
#14822=CARTESIAN_POINT ( 'NONE',  ( 0.1749999999999999889, 7.900000000000000355, 0.4000000000000000222 ) ) ;
#14935=DIRECTION ( 'NONE',  ( -1.000000000000000000, 0.000000000000000000, 1.586032892321649771E-16 ) ) ;
#14938=ORIENTED_EDGE ( 'NONE', *, *, #8937, .T. ) ;
#14942=CARTESIAN_POINT ( 'NONE',  ( -0.1749999999999999889, 9.500000000000000000, 1.600000000000000089 ) ) ;
#14962=PLANE ( 'NONE',  #5099 ) ;
#15026=ORIENTED_EDGE ( 'NONE', *, *, #12870, .T. ) ;
#15068=ORIENTED_EDGE ( 'NONE', *, *, #4570, .F. ) ;
#15100=CARTESIAN_POINT ( 'NONE',  ( -0.1749999999999999889, 9.099999999999999645, 0.4000000000000000222 ) ) ;
#15101=CARTESIAN_POINT ( 'NONE',  ( 0.1749999999999999889, 7.700000000000000178, 0.4000000000000000222 ) ) ;
#15108=VECTOR ( 'NONE', #15879, 1000.000000000000000 ) ;
#15112=DIRECTION ( 'NONE',  ( -1.000000000000000000, 0.000000000000000000, 0.000000000000000000 ) ) ;
#15120=DIRECTION ( 'NONE',  ( -1.000000000000000000, 0.000000000000000000, 0.000000000000000000 ) ) ;
#15122=ORIENTED_EDGE ( 'NONE', *, *, #14488, .T. ) ;
#15138=ORIENTED_EDGE ( 'NONE', *, *, #10737, .F. ) ;
#15202=VECTOR ( 'NONE', #5901, 1000.000000000000000 ) ;
#15207=EDGE_CURVE ( 'NONE', #103, #9728, #6892, .T. ) ;
#15209=ORIENTED_EDGE ( 'NONE', *, *, #15614, .T. ) ;
#15215=ORIENTED_EDGE ( 'NONE', *, *, #16254, .T. ) ;
#15253=CARTESIAN_POINT ( 'NONE',  ( 0.1749999999999999889, 9.099999999999999645, 0.4000000000000000222 ) ) ;
#15274=EDGE_LOOP ( 'NONE', ( #8823, #11872, #16590, #7278, #5638, #3300, #6076, #17435, #6331, #3108, #9461, #40, #17536, #7230, #11487, #953, #13033, #18237 ) ) ;
#15281=ADVANCED_FACE ( 'NONE', ( #3924 ), #5603, .T. ) ;
#15310=LINE ( 'NONE', #11222, #10013 ) ;
#15337=DIRECTION ( 'NONE',  ( -0.000000000000000000, 1.000000000000000000, 0.000000000000000000 ) ) ;
#15369=DIRECTION ( 'NONE',  ( 0.000000000000000000, -2.220446049250309876E-16, 1.000000000000000000 ) ) ;
#15407=CARTESIAN_POINT ( 'NONE',  ( -0.1749999999999999889, 9.500000000000000000, 3.100000000000000089 ) ) ;
#15500=VERTEX_POINT ( 'NONE', #1803 ) ;
#15544=EDGE_CURVE ( 'NONE', #2437, #13650, #17502, .T. ) ;
#15560=LINE ( 'NONE', #537, #4917 ) ;
#15572=CARTESIAN_POINT ( 'NONE',  ( -0.1749999999999999889, 8.200000000000001066, -3.200000000000000178 ) ) ;
#15608=EDGE_CURVE ( 'NONE', #12725, #4752, #12411, .T. ) ;
#15614=EDGE_CURVE ( 'NONE', #6904, #17710, #13354, .T. ) ;
#15615=DIRECTION ( 'NONE',  ( -1.586032892321649771E-16, 0.000000000000000000, -1.000000000000000000 ) ) ;
#15626=EDGE_LOOP ( 'NONE', ( #326, #5386, #3009, #17674 ) ) ;
#15640=VECTOR ( 'NONE', #13340, 1000.000000000000000 ) ;
#15664=VECTOR ( 'NONE', #13692, 1000.000000000000000 ) ;
#15767=ORIENTED_EDGE ( 'NONE', *, *, #13683, .T. ) ;
#15783=LINE ( 'NONE', #3092, #5594 ) ;
#15792=FILL_AREA_STYLE_COLOUR ( '', #18265 ) ;
#15800=EDGE_LOOP ( 'NONE', ( #16288, #11389, #16878, #10971 ) ) ;
#15806=CARTESIAN_POINT ( 'NONE',  ( 0.1749999999999999889, 9.099999999999999645, 0.5999999999999999778 ) ) ;
#15812=( NAMED_UNIT ( * ) SI_UNIT ( $, .STERADIAN. ) SOLID_ANGLE_UNIT ( ) );
#15827=EDGE_CURVE ( 'NONE', #13928, #17154, #15560, .T. ) ;
#15879=DIRECTION ( 'NONE',  ( 6.167905692361979821E-17, 0.000000000000000000, 1.000000000000000000 ) ) ;
#15963=EDGE_LOOP ( 'NONE', ( #1693, #15767, #13296, #4788 ) ) ;
#16003=EDGE_CURVE ( 'NONE', #2052, #15500, #13496, .T. ) ;
#16030=DIRECTION ( 'NONE',  ( 0.000000000000000000, -1.000000000000000000, 2.220446049250320181E-15 ) ) ;
#16036=CARTESIAN_POINT ( 'NONE',  ( 0.1749999999999999889, 9.299999999999998934, 0.4000000000000000222 ) ) ;
#16117=CARTESIAN_POINT ( 'NONE',  ( 0.1749999999999999889, 9.199999999999999289, 0.4000000000000000222 ) ) ;
#16239=VERTEX_POINT ( 'NONE', #16914 ) ;
#16254=EDGE_CURVE ( 'NONE', #17710, #3506, #9975, .T. ) ;
#16263=DIRECTION ( 'NONE',  ( 0.000000000000000000, 0.000000000000000000, -1.000000000000000000 ) ) ;
#16276=LINE ( 'NONE', #915, #15664 ) ;
#16279=ADVANCED_FACE ( 'NONE', ( #7015 ), #14141, .T. ) ;
#16288=ORIENTED_EDGE ( 'NONE', *, *, #6417, .T. ) ;
#16331=LINE ( 'NONE', #8013, #8746 ) ;
#16387=EDGE_CURVE ( 'NONE', #13202, #8663, #17343, .T. ) ;
#16415=PLANE ( 'NONE',  #9413 ) ;
#16429=CARTESIAN_POINT ( 'NONE',  ( 0.1749999999999999889, 7.900000000000000355, 0.5999999999999999778 ) ) ;
#16443=ORIENTED_EDGE ( 'NONE', *, *, #15544, .T. ) ;
#16456=CARTESIAN_POINT ( 'NONE',  ( 0.1749999999999999889, 7.900000000000000355, 0.4000000000000000222 ) ) ;
#16477=DIRECTION ( 'NONE',  ( 0.000000000000000000, -1.000000000000000000, 0.000000000000000000 ) ) ;
#16478=VECTOR ( 'NONE', #11059, 1000.000000000000000 ) ;
#16496=EDGE_CURVE ( 'NONE', #8454, #12005, #5894, .T. ) ;
#16560=VERTEX_POINT ( 'NONE', #16429 ) ;
#16587=ORIENTED_EDGE ( 'NONE', *, *, #16387, .T. ) ;
#16590=ORIENTED_EDGE ( 'NONE', *, *, #2569, .F. ) ;
#16611=CARTESIAN_POINT ( 'NONE',  ( 0.1749999999999999889, 7.799999999999999822, 0.4000000000000000222 ) ) ;
#16637=PLANE ( 'NONE',  #30 ) ;
#16666=CARTESIAN_POINT ( 'NONE',  ( 0.1749999999999999889, 9.099999999999999645, 0.4000000000000000222 ) ) ;
#16684=CARTESIAN_POINT ( 'NONE',  ( 0.1749999999999999889, 9.099999999999999645, 0.4000000000000000222 ) ) ;
#16715=EDGE_CURVE ( 'NONE', #12725, #6904, #9950, .T. ) ;
#16772=LINE ( 'NONE', #1407, #9384 ) ;
#16781=ADVANCED_FACE ( 'NONE', ( #1067 ), #1164, .T. ) ;
#16782=AXIS2_PLACEMENT_3D ( 'NONE', #2826, #15615, #5700 ) ;
#16836=DIRECTION ( 'NONE',  ( 0.000000000000000000, 0.000000000000000000, 1.000000000000000000 ) ) ;
#16878=ORIENTED_EDGE ( 'NONE', *, *, #5071, .F. ) ;
#16914=CARTESIAN_POINT ( 'NONE',  ( 0.1749999999999999889, 9.500000000000000000, 1.600000000000000089 ) ) ;
#16915=ORIENTED_EDGE ( 'NONE', *, *, #4820, .T. ) ;
#16935=CARTESIAN_POINT ( 'NONE',  ( 0.1749999999999999889, 7.500000000000000000, 1.600000000000000089 ) ) ;
#16953=AXIS2_PLACEMENT_3D ( 'NONE', #15806, #3112, #8764 ) ;
#16967=EDGE_CURVE ( 'NONE', #13610, #8454, #8939, .T. ) ;
#17005=ORIENTED_EDGE ( 'NONE', *, *, #15827, .T. ) ;
#17035=CARTESIAN_POINT ( 'NONE',  ( 0.1749999999999999889, 7.500000000000000000, 3.100000000000000089 ) ) ;
#17091=DIRECTION ( 'NONE',  ( -1.000000000000000000, 0.000000000000000000, 6.123233995736769734E-17 ) ) ;
#17094=EDGE_LOOP ( 'NONE', ( #3015, #9521, #1563, #3517 ) ) ;
#17118=ORIENTED_EDGE ( 'NONE', *, *, #4307, .F. ) ;
#17153=EDGE_CURVE ( 'NONE', #16560, #2052, #2181, .T. ) ;
#17154=VERTEX_POINT ( 'NONE', #13469 ) ;
#17176=PLANE ( 'NONE',  #16953 ) ;
#17237=LINE ( 'NONE', #16117, #14671 ) ;
#17240=SURFACE_STYLE_FILL_AREA ( #4559 ) ;
#17304=VERTEX_POINT ( 'NONE', #1255 ) ;
#17313=EDGE_LOOP ( 'NONE', ( #16587, #14938, #10481, #10084 ) ) ;
#17317=ORIENTED_EDGE ( 'NONE', *, *, #16967, .F. ) ;
#17343=LINE ( 'NONE', #4568, #18238 ) ;
#17389=EDGE_CURVE ( 'NONE', #1389, #103, #11348, .T. ) ;
#17402=LINE ( 'NONE', #16036, #1467 ) ;
#17418=DIRECTION ( 'NONE',  ( -1.000000000000000000, 0.000000000000000000, 0.000000000000000000 ) ) ;
#17435=ORIENTED_EDGE ( 'NONE', *, *, #11852, .F. ) ;
#17483=CARTESIAN_POINT ( 'NONE',  ( 0.1749999999999999889, 7.500000000000000000, 1.600000000000000089 ) ) ;
#17502=LINE ( 'NONE', #11797, #7577 ) ;
#17536=ORIENTED_EDGE ( 'NONE', *, *, #6417, .F. ) ;
#17563=DIRECTION ( 'NONE',  ( 0.000000000000000000, 0.000000000000000000, -1.000000000000000000 ) ) ;
#17605=VECTOR ( 'NONE', #1333, 1000.000000000000000 ) ;
#17608=CARTESIAN_POINT ( 'NONE',  ( 0.1749999999999999889, 7.900000000000000355, 0.5999999999999999778 ) ) ;
#17668=VECTOR ( 'NONE', #13651, 1000.000000000000000 ) ;
#17674=ORIENTED_EDGE ( 'NONE', *, *, #17153, .F. ) ;
#17681=AXIS2_PLACEMENT_3D ( 'NONE', #11191, #16836, #4146 ) ;
#17710=VERTEX_POINT ( 'NONE', #18086 ) ;
#17742=LINE ( 'NONE', #10632, #4978 ) ;
#17743=DIRECTION ( 'NONE',  ( 6.938893903907229610E-17, 0.000000000000000000, 1.000000000000000000 ) ) ;
#17762=CARTESIAN_POINT ( 'NONE',  ( -0.1749999999999999889, 7.700000000000000178, 0.4000000000000000222 ) ) ;
#17796=DIRECTION ( 'NONE',  ( 9.251858538542969116E-17, 0.000000000000000000, 1.000000000000000000 ) ) ;
#17812=PLANE ( 'NONE',  #4347 ) ;
#17822=PLANE ( 'NONE',  #2030 ) ;
#17844=EDGE_CURVE ( 'NONE', #13844, #11906, #5320, .T. ) ;
#17856=ORIENTED_EDGE ( 'NONE', *, *, #2569, .T. ) ;
#17867=ADVANCED_FACE ( 'NONE', ( #10867 ), #16415, .T. ) ;
#17886=CARTESIAN_POINT ( 'NONE',  ( 0.1749999999999999889, 9.500000000000000000, 3.100000000000000089 ) ) ;
#17895=CARTESIAN_POINT ( 'NONE',  ( 0.1749999999999999889, 7.500000000000000000, 1.600000000000000089 ) ) ;
#17912=CARTESIAN_POINT ( 'NONE',  ( -0.1749999999999999889, 7.500000000000000000, 3.100000000000000089 ) ) ;
#17953=VECTOR ( 'NONE', #9867, 1000.000000000000000 ) ;
#17967=VERTEX_POINT ( 'NONE', #5490 ) ;
#17986=VECTOR ( 'NONE', #6350, 1000.000000000000000 ) ;
#17999=EDGE_CURVE ( 'NONE', #16239, #17967, #3081, .T. ) ;
#18045=ORIENTED_EDGE ( 'NONE', *, *, #16496, .T. ) ;
#18086=CARTESIAN_POINT ( 'NONE',  ( 0.1749999999999999889, 8.800000000000000711, 0.4000000000000000222 ) ) ;
#18087=CARTESIAN_POINT ( 'NONE',  ( 0.1749999999999999889, 7.900000000000000355, 0.5999999999999999778 ) ) ;
#18098=CARTESIAN_POINT ( 'NONE',  ( 0.1749999999999999889, 9.299999999999998934, 1.600000000000000089 ) ) ;
#18125=CARTESIAN_POINT ( 'NONE',  ( -0.1749999999999999889, 9.299999999999998934, 1.600000000000000089 ) ) ;
#18237=ORIENTED_EDGE ( 'NONE', *, *, #9005, .F. ) ;
#18238=VECTOR ( 'NONE', #5980, 1000.000000000000000 ) ;
#18254=VECTOR ( 'NONE', #2273, 1000.000000000000000 ) ;
#18255=ADVANCED_FACE ( 'NONE', ( #12239 ), #7031, .T. ) ;
#18265=COLOUR_RGB ( '', 0.66274510, 0.83137255, 0.94901961) ;
ENDSEC;
END-ISO-10303-21;
